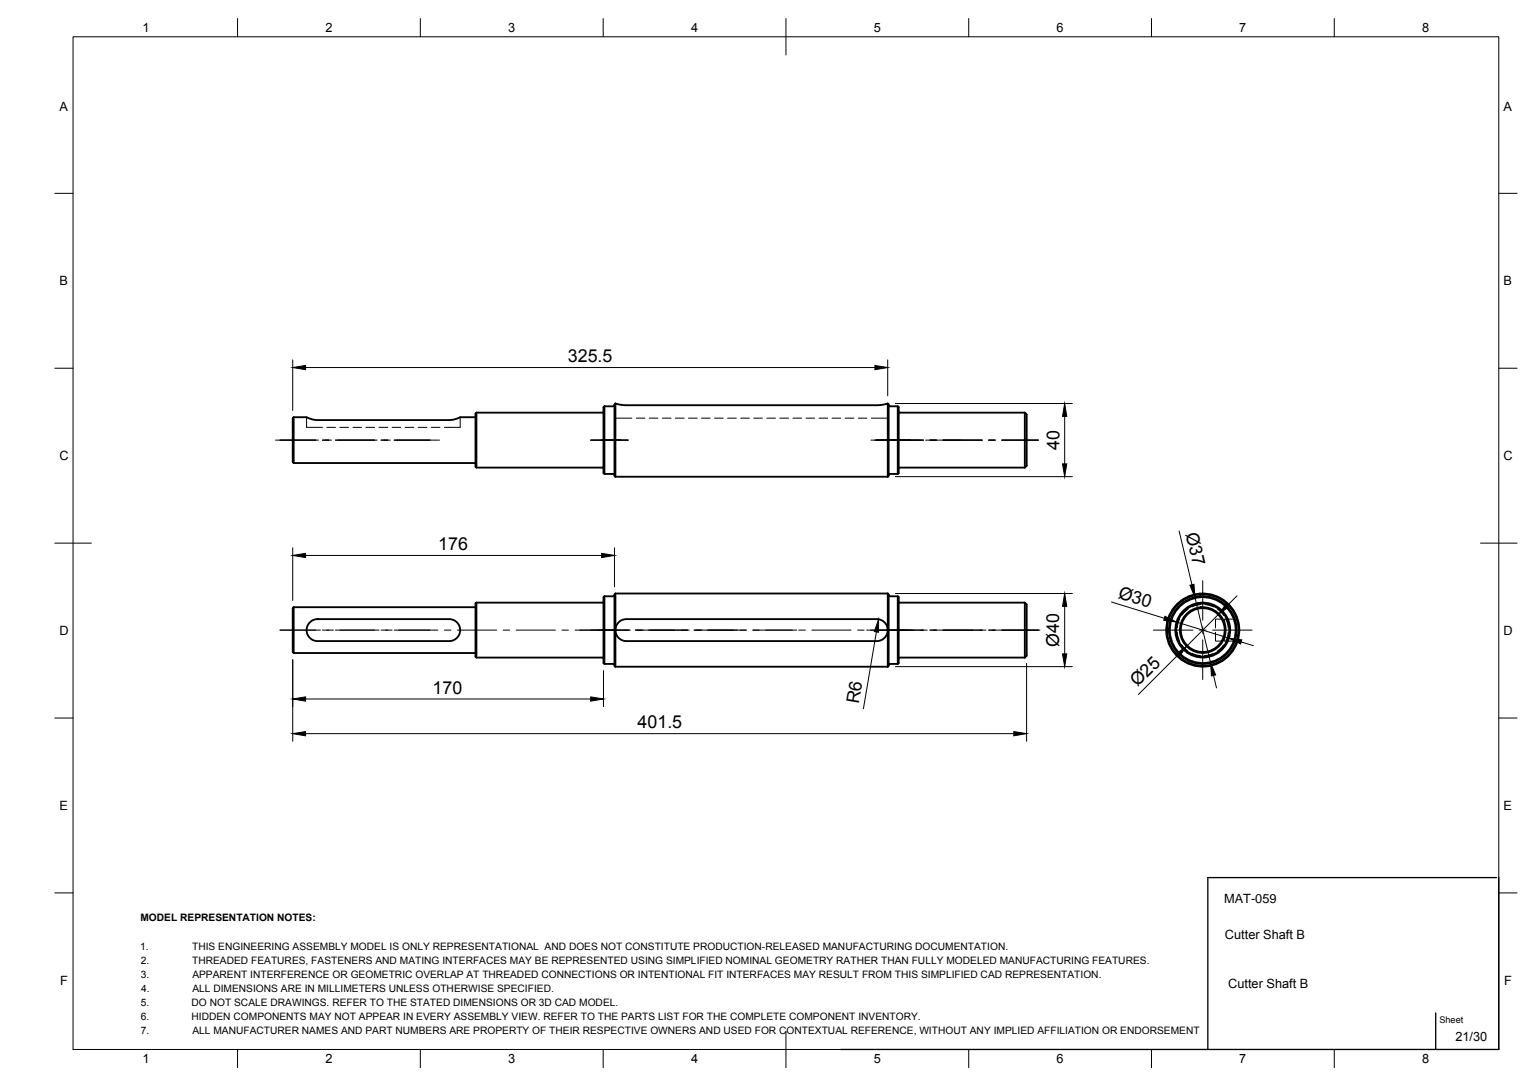
ISO-10303-21;
HEADER;
/* Generated by software containing ST-Developer
 * from STEP Tools, Inc. (www.steptools.com) 
 */

FILE_DESCRIPTION(
/* description */ ('', 'CAx-IF Rec.Pracs.---Representation and Presentation of Product Manufa
cturing Information (PMI)---4.0---2014-10-13'),
/* implementation_level */ '2;1');

FILE_NAME(
/* name */ 'Cutter Shaft B.step',
/* time_stamp */ '2026-10-28T23:00:48+01:00',
/* author */ (''),
/* organization */ (''),
/* preprocessor_version */ 'ST-DEVELOPER v20.2',
/* originating_system */ 'Autodesk Translation Framework v15.17.0.0',
/* authorisation */ '');

FILE_SCHEMA (('AP242_MANAGED_MODEL_BASED_3D_ENGINEERING_MIM_LF { 1 0 10303 442 2 1 4 }'));
ENDSEC;

DATA;
#10=MECHANICAL_DESIGN_GEOMETRIC_PRESENTATION_REPRESENTATION('',(#993),#61811);
#609=CONICAL_SURFACE('',#36036,12.25,0.785398163397429);
#610=CONICAL_SURFACE('',#36043,14.75,0.785398163397442);
#611=CONICAL_SURFACE('',#36058,18.25,0.785398163397442);
#612=CONICAL_SURFACE('',#36079,18.25,0.78539816339745);
#613=CONICAL_SURFACE('',#36085,14.5,0.785398163397445);
#614=CONICAL_SURFACE('',#36103,19.75,0.78539816339745);
#615=CONICAL_SURFACE('',#36104,19.75,0.78539816339745);
#825=B_SPLINE_CURVE_WITH_KNOTS('',3,(#56114,#56115,#56116,#56117,#56118,
#56119,#56120,#56121,#56122,#56123),.UNSPECIFIED.,.F.,.F.,(4,2,2,2,4),(0.910129823137503,
1.1376283823127,1.36512694148791,1.59269329388146,1.82025964627501),
 .UNSPECIFIED.);
#826=B_SPLINE_CURVE_WITH_KNOTS('',3,(#56127,#56128,#56129,#56130,#56131,
#56132,#56133,#56134,#56135,#56136),.UNSPECIFIED.,.F.,.F.,(4,2,2,2,4),(1.82025964627501,
2.04782599866856,2.27539235106211,2.50289091023731,2.73038946941251),
 .UNSPECIFIED.);
#827=B_SPLINE_CURVE_WITH_KNOTS('',3,(#56154,#56155,#56156,#56157,#56158,
#56159,#56160,#56161,#56162,#56163,#56164,#56165,#56166,#56167,#56168,#56169,
#56170,#56171),.UNSPECIFIED.,.F.,.F.,(4,2,2,2,2,2,2,2,4),(-1.84177286144596,
-1.6112902776922,-1.38080769393844,-1.15084706233071,-0.920886430722982,
-0.690925799115252,-0.460965167507522,-0.230482583753761,0.),
 .UNSPECIFIED.);
#828=B_SPLINE_CURVE_WITH_KNOTS('',3,(#56174,#56175,#56176,#56177,#56178,
#56179,#56180,#56181,#56182,#56183,#56184,#56185,#56186,#56187,#56188,#56189,
#56190,#56191),.UNSPECIFIED.,.F.,.F.,(4,2,2,2,2,2,2,2,4),(-3.68354572289192,
-3.45306313913815,-3.22258055538439,-2.99261992377667,-2.76265929216894,
-2.53269866056121,-2.30273802895348,-2.07225544519972,-1.84177286144596),
 .UNSPECIFIED.);
#829=B_SPLINE_CURVE_WITH_KNOTS('',3,(#56285,#56286,#56287,#56288,#56289,
#56290,#56291,#56292,#56293,#56294),.UNSPECIFIED.,.F.,.F.,(4,2,2,2,4),(2.73038946941251,
2.95788802858771,3.18538658776291,3.41295294015646,3.64051929255001),
 .UNSPECIFIED.);
#830=B_SPLINE_CURVE_WITH_KNOTS('',3,(#56306,#56307,#56308,#56309,#56310,
#56311,#56312,#56313,#56314,#56315),.UNSPECIFIED.,.F.,.F.,(4,2,2,2,4),(0.,
0.22756635239355,0.4551327047871,0.682631263962301,0.910129823137503),
 .UNSPECIFIED.);
#902=TOROIDAL_SURFACE('',#36067,15.5,0.5);
#903=TOROIDAL_SURFACE('',#36074,15.5,0.5);
#904=TOROIDAL_SURFACE('',#36098,19.,0.500000000000029);
#905=TOROIDAL_SURFACE('',#36108,19.,0.499999999999998);
#929=SHAPE_REPRESENTATION_RELATIONSHIP('SRR','None',#61989,#954);
#954=ADVANCED_BREP_SHAPE_REPRESENTATION('',(#1032),#61802);
#993=STYLED_ITEM('',(#62156),#1032);
#1032=MANIFOLD_SOLID_BREP('Body1',#33823);
#1380=CYLINDRICAL_SURFACE('',#36033,20.);
#1381=CYLINDRICAL_SURFACE('',#36040,12.5);
#1382=CYLINDRICAL_SURFACE('',#36047,15.);
#1383=CYLINDRICAL_SURFACE('',#36052,5.99999999999999);
#1384=CYLINDRICAL_SURFACE('',#36055,6.00000000000001);
#1385=CYLINDRICAL_SURFACE('',#36064,18.5);
#1386=CYLINDRICAL_SURFACE('',#36071,15.);
#1387=CYLINDRICAL_SURFACE('',#36082,18.5);
#1388=CYLINDRICAL_SURFACE('',#36088,6.);
#1389=CYLINDRICAL_SURFACE('',#36092,6.);
#1390=CYLINDRICAL_SURFACE('',#36095,20.);
#2121=FACE_BOUND('',#7350,.T.);
#2122=FACE_BOUND('',#7355,.T.);
#2123=FACE_BOUND('',#7363,.T.);
#2124=FACE_BOUND('',#7369,.T.);
#2125=FACE_BOUND('',#7382,.T.);
#2126=FACE_BOUND('',#7386,.T.);
#3075=CIRCLE('',#36034,20.);
#3076=CIRCLE('',#36035,20.);
#3077=CIRCLE('',#36037,12.5);
#3078=CIRCLE('',#36038,12.5);
#3079=CIRCLE('',#36039,12.);
#3080=CIRCLE('',#36041,12.5);
#3081=CIRCLE('',#36044,15.);
#3082=CIRCLE('',#36045,15.);
#3083=CIRCLE('',#36046,14.5);
#3084=CIRCLE('',#36048,15.);
#3085=CIRCLE('',#36049,15.);
#3086=CIRCLE('',#36053,5.99999999999999);
#3087=CIRCLE('',#36056,6.00000000000001);
#3088=CIRCLE('',#36059,18.5);
#3089=CIRCLE('',#36060,18.5);
#3090=CIRCLE('',#36061,18.);
#3091=CIRCLE('',#36063,15.5);
#3092=CIRCLE('',#36065,18.5);
#3093=CIRCLE('',#36066,18.5);
#3094=CIRCLE('',#36068,0.5);
#3095=CIRCLE('',#36069,15.);
#3096=CIRCLE('',#36070,15.);
#3097=CIRCLE('',#36072,15.);
#3098=CIRCLE('',#36073,15.);
#3099=CIRCLE('',#36075,0.5);
#3100=CIRCLE('',#36076,15.5);
#3101=CIRCLE('',#36078,18.);
#3102=CIRCLE('',#36080,18.5);
#3103=CIRCLE('',#36081,18.5);
#3104=CIRCLE('',#36083,18.5);
#3105=CIRCLE('',#36084,18.5);
#3106=CIRCLE('',#36086,14.);
#3107=CIRCLE('',#36089,6.);
#3108=CIRCLE('',#36093,6.);
#3109=CIRCLE('',#36096,20.);
#3110=CIRCLE('',#36097,20.);
#3111=CIRCLE('',#36099,19.);
#3112=CIRCLE('',#36100,0.500000000000029);
#3113=CIRCLE('',#36102,19.5);
#3114=CIRCLE('',#36105,19.5);
#3115=CIRCLE('',#36107,19.);
#3116=CIRCLE('',#36109,0.499999999999998);
#5226=FACE_OUTER_BOUND('',#7347,.T.);
#5227=FACE_OUTER_BOUND('',#7348,.T.);
#5228=FACE_OUTER_BOUND('',#7349,.T.);
#5229=FACE_OUTER_BOUND('',#7351,.T.);
#5230=FACE_OUTER_BOUND('',#7352,.T.);
#5231=FACE_OUTER_BOUND('',#7353,.T.);
#5232=FACE_OUTER_BOUND('',#7354,.T.);
#5233=FACE_OUTER_BOUND('',#7356,.T.);
#5234=FACE_OUTER_BOUND('',#7357,.T.);
#5235=FACE_OUTER_BOUND('',#7358,.T.);
#5236=FACE_OUTER_BOUND('',#7359,.T.);
#5237=FACE_OUTER_BOUND('',#7360,.T.);
#5238=FACE_OUTER_BOUND('',#7361,.T.);
#5239=FACE_OUTER_BOUND('',#7362,.T.);
#5240=FACE_OUTER_BOUND('',#7364,.T.);
#5241=FACE_OUTER_BOUND('',#7365,.T.);
#5242=FACE_OUTER_BOUND('',#7366,.T.);
#5243=FACE_OUTER_BOUND('',#7367,.T.);
#5244=FACE_OUTER_BOUND('',#7368,.T.);
#5245=FACE_OUTER_BOUND('',#7370,.T.);
#5246=FACE_OUTER_BOUND('',#7371,.T.);
#5247=FACE_OUTER_BOUND('',#7372,.T.);
#5248=FACE_OUTER_BOUND('',#7373,.T.);
#5249=FACE_OUTER_BOUND('',#7374,.T.);
#5250=FACE_OUTER_BOUND('',#7375,.T.);
#5251=FACE_OUTER_BOUND('',#7376,.T.);
#5252=FACE_OUTER_BOUND('',#7377,.T.);
#5253=FACE_OUTER_BOUND('',#7378,.T.);
#5254=FACE_OUTER_BOUND('',#7379,.T.);
#5255=FACE_OUTER_BOUND('',#7380,.T.);
#5256=FACE_OUTER_BOUND('',#7381,.T.);
#5257=FACE_OUTER_BOUND('',#7383,.T.);
#5258=FACE_OUTER_BOUND('',#7384,.T.);
#5259=FACE_OUTER_BOUND('',#7385,.T.);
#5260=FACE_OUTER_BOUND('',#7387,.T.);
#7347=EDGE_LOOP('',(#26382,#26383,#26384,#26385,#26386,#26387));
#7348=EDGE_LOOP('',(#26388,#26389,#26390,#26391,#26392));
#7349=EDGE_LOOP('',(#26393,#26394,#26395,#26396,#26397));
#7350=EDGE_LOOP('',(#26398,#26399,#26400,#26401));
#7351=EDGE_LOOP('',(#26402));
#7352=EDGE_LOOP('',(#26403,#26404,#26405,#26406,#26407));
#7353=EDGE_LOOP('',(#26408,#26409,#26410,#26411,#26412,#26413));
#7354=EDGE_LOOP('',(#26414));
#7355=EDGE_LOOP('',(#26415));
#7356=EDGE_LOOP('',(#26416,#26417,#26418,#26419));
#7357=EDGE_LOOP('',(#26420,#26421,#26422,#26423));
#7358=EDGE_LOOP('',(#26424,#26425,#26426,#26427));
#7359=EDGE_LOOP('',(#26428,#26429,#26430,#26431));
#7360=EDGE_LOOP('',(#26432,#26433,#26434,#26435));
#7361=EDGE_LOOP('',(#26436,#26437,#26438,#26439,#26440));
#7362=EDGE_LOOP('',(#26441));
#7363=EDGE_LOOP('',(#26442));
#7364=EDGE_LOOP('',(#26443,#26444,#26445,#26446,#26447,#26448));
#7365=EDGE_LOOP('',(#26449,#26450,#26451,#26452,#26453));
#7366=EDGE_LOOP('',(#26454,#26455,#26456,#26457,#26458,#26459));
#7367=EDGE_LOOP('',(#26460,#26461,#26462,#26463,#26464));
#7368=EDGE_LOOP('',(#26465));
#7369=EDGE_LOOP('',(#26466));
#7370=EDGE_LOOP('',(#26467,#26468,#26469,#26470,#26471));
#7371=EDGE_LOOP('',(#26472,#26473,#26474,#26475,#26476,#26477));
#7372=EDGE_LOOP('',(#26478,#26479,#26480,#26481,#26482));
#7373=EDGE_LOOP('',(#26483));
#7374=EDGE_LOOP('',(#26484,#26485,#26486,#26487,#26488));
#7375=EDGE_LOOP('',(#26489,#26490,#26491,#26492));
#7376=EDGE_LOOP('',(#26493,#26494,#26495,#26496));
#7377=EDGE_LOOP('',(#26497,#26498,#26499,#26500,#26501));
#7378=EDGE_LOOP('',(#26502,#26503,#26504,#26505));
#7379=EDGE_LOOP('',(#26506,#26507,#26508,#26509,#26510,#26511));
#7380=EDGE_LOOP('',(#26512,#26513,#26514,#26515,#26516));
#7381=EDGE_LOOP('',(#26517));
#7382=EDGE_LOOP('',(#26518));
#7383=EDGE_LOOP('',(#26519,#26520,#26521,#26522,#26523));
#7384=EDGE_LOOP('',(#26524,#26525,#26526,#26527,#26528));
#7385=EDGE_LOOP('',(#26529));
#7386=EDGE_LOOP('',(#26530));
#7387=EDGE_LOOP('',(#26531,#26532,#26533,#26534,#26535));
#9784=LINE('',#56110,#12331);
#9785=LINE('',#56125,#12332);
#9786=LINE('',#56144,#12333);
#9787=LINE('',#56148,#12334);
#9788=LINE('',#56152,#12335);
#9789=LINE('',#56173,#12336);
#9790=LINE('',#56199,#12337);
#9791=LINE('',#56203,#12338);
#9792=LINE('',#56210,#12339);
#9793=LINE('',#56212,#12340);
#9794=LINE('',#56213,#12341);
#9795=LINE('',#56217,#12342);
#9796=LINE('',#56220,#12343);
#9797=LINE('',#56221,#12344);
#9798=LINE('',#56231,#12345);
#9799=LINE('',#56240,#12346);
#9800=LINE('',#56250,#12347);
#9801=LINE('',#56266,#12348);
#9802=LINE('',#56269,#12349);
#9803=LINE('',#56275,#12350);
#9804=LINE('',#56280,#12351);
#9805=LINE('',#56284,#12352);
#9806=LINE('',#56297,#12353);
#9807=LINE('',#56299,#12354);
#9808=LINE('',#56300,#12355);
#9809=LINE('',#56303,#12356);
#9810=LINE('',#56304,#12357);
#9811=LINE('',#56329,#12358);
#9812=LINE('',#56332,#12359);
#12331=VECTOR('',#43448,20.);
#12332=VECTOR('',#43451,10.);
#12333=VECTOR('',#43460,12.25);
#12334=VECTOR('',#43465,12.5);
#12335=VECTOR('',#43468,10.);
#12336=VECTOR('',#43469,10.);
#12337=VECTOR('',#43478,14.75);
#12338=VECTOR('',#43483,15.);
#12339=VECTOR('',#43492,10.);
#12340=VECTOR('',#43493,10.);
#12341=VECTOR('',#43494,10.);
#12342=VECTOR('',#43499,10.);
#12343=VECTOR('',#43502,10.);
#12344=VECTOR('',#43503,10.);
#12345=VECTOR('',#43516,18.25);
#12346=VECTOR('',#43527,18.5);
#12347=VECTOR('',#43540,15.);
#12348=VECTOR('',#43561,18.25);
#12349=VECTOR('',#43564,18.5);
#12350=VECTOR('',#43571,14.5);
#12351=VECTOR('',#43578,10.);
#12352=VECTOR('',#43581,10.);
#12353=VECTOR('',#43584,10.);
#12354=VECTOR('',#43585,10.);
#12355=VECTOR('',#43586,10.);
#12356=VECTOR('',#43589,10.);
#12357=VECTOR('',#43590,10.);
#12358=VECTOR('',#43615,19.75);
#12359=VECTOR('',#43618,19.75);
#15047=VERTEX_POINT('',#56108);
#15048=VERTEX_POINT('',#56109);
#15049=VERTEX_POINT('',#56111);
#15050=VERTEX_POINT('',#56113);
#15051=VERTEX_POINT('',#56124);
#15052=VERTEX_POINT('',#56126);
#15053=VERTEX_POINT('',#56139);
#15054=VERTEX_POINT('',#56140);
#15055=VERTEX_POINT('',#56143);
#15056=VERTEX_POINT('',#56147);
#15057=VERTEX_POINT('',#56150);
#15058=VERTEX_POINT('',#56151);
#15059=VERTEX_POINT('',#56153);
#15060=VERTEX_POINT('',#56172);
#15061=VERTEX_POINT('',#56194);
#15062=VERTEX_POINT('',#56195);
#15063=VERTEX_POINT('',#56198);
#15064=VERTEX_POINT('',#56202);
#15065=VERTEX_POINT('',#56204);
#15066=VERTEX_POINT('',#56209);
#15067=VERTEX_POINT('',#56211);
#15068=VERTEX_POINT('',#56215);
#15069=VERTEX_POINT('',#56219);
#15070=VERTEX_POINT('',#56226);
#15071=VERTEX_POINT('',#56227);
#15072=VERTEX_POINT('',#56230);
#15073=VERTEX_POINT('',#56234);
#15074=VERTEX_POINT('',#56237);
#15075=VERTEX_POINT('',#56238);
#15076=VERTEX_POINT('',#56243);
#15077=VERTEX_POINT('',#56245);
#15078=VERTEX_POINT('',#56249);
#15079=VERTEX_POINT('',#56251);
#15080=VERTEX_POINT('',#56255);
#15081=VERTEX_POINT('',#56259);
#15082=VERTEX_POINT('',#56262);
#15083=VERTEX_POINT('',#56263);
#15084=VERTEX_POINT('',#56268);
#15085=VERTEX_POINT('',#56270);
#15086=VERTEX_POINT('',#56274);
#15087=VERTEX_POINT('',#56279);
#15088=VERTEX_POINT('',#56281);
#15089=VERTEX_POINT('',#56283);
#15090=VERTEX_POINT('',#56296);
#15091=VERTEX_POINT('',#56298);
#15092=VERTEX_POINT('',#56302);
#15093=VERTEX_POINT('',#56322);
#15094=VERTEX_POINT('',#56326);
#15095=VERTEX_POINT('',#56331);
#15096=VERTEX_POINT('',#56335);
#19093=EDGE_CURVE('',#15047,#15048,#9784,.T.);
#19094=EDGE_CURVE('',#15049,#15047,#3075,.T.);
#19095=EDGE_CURVE('',#15049,#15050,#825,.T.);
#19096=EDGE_CURVE('',#15050,#15051,#9785,.T.);
#19097=EDGE_CURVE('',#15051,#15052,#826,.T.);
#19098=EDGE_CURVE('',#15052,#15048,#3076,.T.);
#19099=EDGE_CURVE('',#15053,#15054,#3077,.T.);
#19100=EDGE_CURVE('',#15054,#15053,#3078,.T.);
#19101=EDGE_CURVE('',#15053,#15055,#9786,.T.);
#19102=EDGE_CURVE('',#15055,#15055,#3079,.T.);
#19103=EDGE_CURVE('',#15054,#15056,#9787,.T.);
#19104=EDGE_CURVE('',#15056,#15056,#3080,.T.);
#19105=EDGE_CURVE('',#15057,#15058,#9788,.T.);
#19106=EDGE_CURVE('',#15058,#15059,#827,.T.);
#19107=EDGE_CURVE('',#15059,#15060,#9789,.T.);
#19108=EDGE_CURVE('',#15060,#15057,#828,.T.);
#19109=EDGE_CURVE('',#15061,#15062,#3081,.T.);
#19110=EDGE_CURVE('',#15062,#15061,#3082,.T.);
#19111=EDGE_CURVE('',#15061,#15063,#9790,.T.);
#19112=EDGE_CURVE('',#15063,#15063,#3083,.T.);
#19113=EDGE_CURVE('',#15062,#15064,#9791,.T.);
#19114=EDGE_CURVE('',#15065,#15064,#3084,.T.);
#19115=EDGE_CURVE('',#15064,#15065,#3085,.T.);
#19116=EDGE_CURVE('',#15059,#15066,#9792,.T.);
#19117=EDGE_CURVE('',#15066,#15067,#9793,.T.);
#19118=EDGE_CURVE('',#15060,#15067,#9794,.T.);
#19119=EDGE_CURVE('',#15067,#15068,#3086,.T.);
#19120=EDGE_CURVE('',#15057,#15068,#9795,.T.);
#19121=EDGE_CURVE('',#15068,#15069,#9796,.T.);
#19122=EDGE_CURVE('',#15058,#15069,#9797,.T.);
#19123=EDGE_CURVE('',#15069,#15066,#3087,.T.);
#19124=EDGE_CURVE('',#15070,#15071,#3088,.T.);
#19125=EDGE_CURVE('',#15071,#15070,#3089,.T.);
#19126=EDGE_CURVE('',#15070,#15072,#9798,.T.);
#19127=EDGE_CURVE('',#15072,#15072,#3090,.T.);
#19128=EDGE_CURVE('',#15073,#15073,#3091,.T.);
#19129=EDGE_CURVE('',#15074,#15075,#3092,.T.);
#19130=EDGE_CURVE('',#15074,#15071,#9799,.T.);
#19131=EDGE_CURVE('',#15075,#15074,#3093,.T.);
#19132=EDGE_CURVE('',#15073,#15076,#3094,.T.);
#19133=EDGE_CURVE('',#15076,#15077,#3095,.T.);
#19134=EDGE_CURVE('',#15077,#15076,#3096,.T.);
#19135=EDGE_CURVE('',#15077,#15078,#9800,.T.);
#19136=EDGE_CURVE('',#15079,#15078,#3097,.T.);
#19137=EDGE_CURVE('',#15078,#15079,#3098,.T.);
#19138=EDGE_CURVE('',#15065,#15080,#3099,.T.);
#19139=EDGE_CURVE('',#15080,#15080,#3100,.T.);
#19140=EDGE_CURVE('',#15081,#15081,#3101,.T.);
#19141=EDGE_CURVE('',#15082,#15083,#3102,.T.);
#19142=EDGE_CURVE('',#15083,#15082,#3103,.T.);
#19143=EDGE_CURVE('',#15082,#15081,#9801,.T.);
#19144=EDGE_CURVE('',#15083,#15084,#9802,.T.);
#19145=EDGE_CURVE('',#15084,#15085,#3104,.T.);
#19146=EDGE_CURVE('',#15085,#15084,#3105,.T.);
#19147=EDGE_CURVE('',#15079,#15086,#9803,.T.);
#19148=EDGE_CURVE('',#15086,#15086,#3106,.T.);
#19149=EDGE_CURVE('',#15051,#15087,#9804,.T.);
#19150=EDGE_CURVE('',#15087,#15088,#3107,.T.);
#19151=EDGE_CURVE('',#15089,#15088,#9805,.T.);
#19152=EDGE_CURVE('',#15052,#15089,#829,.T.);
#19153=EDGE_CURVE('',#15089,#15090,#9806,.T.);
#19154=EDGE_CURVE('',#15088,#15091,#9807,.T.);
#19155=EDGE_CURVE('',#15090,#15091,#9808,.T.);
#19156=EDGE_CURVE('',#15050,#15092,#9809,.T.);
#19157=EDGE_CURVE('',#15092,#15087,#9810,.T.);
#19158=EDGE_CURVE('',#15090,#15049,#830,.T.);
#19159=EDGE_CURVE('',#15091,#15092,#3108,.T.);
#19160=EDGE_CURVE('',#15048,#15052,#3109,.T.);
#19161=EDGE_CURVE('',#15047,#15049,#3110,.T.);
#19162=EDGE_CURVE('',#15093,#15093,#3111,.T.);
#19163=EDGE_CURVE('',#15093,#15075,#3112,.T.);
#19164=EDGE_CURVE('',#15094,#15094,#3113,.T.);
#19165=EDGE_CURVE('',#15048,#15094,#9811,.T.);
#19166=EDGE_CURVE('',#15047,#15095,#9812,.T.);
#19167=EDGE_CURVE('',#15095,#15095,#3114,.T.);
#19168=EDGE_CURVE('',#15096,#15096,#3115,.T.);
#19169=EDGE_CURVE('',#15085,#15096,#3116,.T.);
#26382=ORIENTED_EDGE('',*,*,#19093,.F.);
#26383=ORIENTED_EDGE('',*,*,#19094,.F.);
#26384=ORIENTED_EDGE('',*,*,#19095,.T.);
#26385=ORIENTED_EDGE('',*,*,#19096,.T.);
#26386=ORIENTED_EDGE('',*,*,#19097,.T.);
#26387=ORIENTED_EDGE('',*,*,#19098,.T.);
#26388=ORIENTED_EDGE('',*,*,#19099,.T.);
#26389=ORIENTED_EDGE('',*,*,#19100,.T.);
#26390=ORIENTED_EDGE('',*,*,#19101,.T.);
#26391=ORIENTED_EDGE('',*,*,#19102,.T.);
#26392=ORIENTED_EDGE('',*,*,#19101,.F.);
#26393=ORIENTED_EDGE('',*,*,#19099,.F.);
#26394=ORIENTED_EDGE('',*,*,#19100,.F.);
#26395=ORIENTED_EDGE('',*,*,#19103,.T.);
#26396=ORIENTED_EDGE('',*,*,#19104,.T.);
#26397=ORIENTED_EDGE('',*,*,#19103,.F.);
#26398=ORIENTED_EDGE('',*,*,#19105,.T.);
#26399=ORIENTED_EDGE('',*,*,#19106,.T.);
#26400=ORIENTED_EDGE('',*,*,#19107,.T.);
#26401=ORIENTED_EDGE('',*,*,#19108,.T.);
#26402=ORIENTED_EDGE('',*,*,#19102,.F.);
#26403=ORIENTED_EDGE('',*,*,#19109,.T.);
#26404=ORIENTED_EDGE('',*,*,#19110,.T.);
#26405=ORIENTED_EDGE('',*,*,#19111,.T.);
#26406=ORIENTED_EDGE('',*,*,#19112,.T.);
#26407=ORIENTED_EDGE('',*,*,#19111,.F.);
#26408=ORIENTED_EDGE('',*,*,#19109,.F.);
#26409=ORIENTED_EDGE('',*,*,#19110,.F.);
#26410=ORIENTED_EDGE('',*,*,#19113,.T.);
#26411=ORIENTED_EDGE('',*,*,#19114,.F.);
#26412=ORIENTED_EDGE('',*,*,#19115,.F.);
#26413=ORIENTED_EDGE('',*,*,#19113,.F.);
#26414=ORIENTED_EDGE('',*,*,#19112,.F.);
#26415=ORIENTED_EDGE('',*,*,#19104,.F.);
#26416=ORIENTED_EDGE('',*,*,#19107,.F.);
#26417=ORIENTED_EDGE('',*,*,#19116,.T.);
#26418=ORIENTED_EDGE('',*,*,#19117,.T.);
#26419=ORIENTED_EDGE('',*,*,#19118,.F.);
#26420=ORIENTED_EDGE('',*,*,#19108,.F.);
#26421=ORIENTED_EDGE('',*,*,#19118,.T.);
#26422=ORIENTED_EDGE('',*,*,#19119,.T.);
#26423=ORIENTED_EDGE('',*,*,#19120,.F.);
#26424=ORIENTED_EDGE('',*,*,#19105,.F.);
#26425=ORIENTED_EDGE('',*,*,#19120,.T.);
#26426=ORIENTED_EDGE('',*,*,#19121,.T.);
#26427=ORIENTED_EDGE('',*,*,#19122,.F.);
#26428=ORIENTED_EDGE('',*,*,#19106,.F.);
#26429=ORIENTED_EDGE('',*,*,#19122,.T.);
#26430=ORIENTED_EDGE('',*,*,#19123,.T.);
#26431=ORIENTED_EDGE('',*,*,#19116,.F.);
#26432=ORIENTED_EDGE('',*,*,#19123,.F.);
#26433=ORIENTED_EDGE('',*,*,#19121,.F.);
#26434=ORIENTED_EDGE('',*,*,#19119,.F.);
#26435=ORIENTED_EDGE('',*,*,#19117,.F.);
#26436=ORIENTED_EDGE('',*,*,#19124,.T.);
#26437=ORIENTED_EDGE('',*,*,#19125,.T.);
#26438=ORIENTED_EDGE('',*,*,#19126,.T.);
#26439=ORIENTED_EDGE('',*,*,#19127,.T.);
#26440=ORIENTED_EDGE('',*,*,#19126,.F.);
#26441=ORIENTED_EDGE('',*,*,#19127,.F.);
#26442=ORIENTED_EDGE('',*,*,#19128,.F.);
#26443=ORIENTED_EDGE('',*,*,#19129,.F.);
#26444=ORIENTED_EDGE('',*,*,#19130,.T.);
#26445=ORIENTED_EDGE('',*,*,#19124,.F.);
#26446=ORIENTED_EDGE('',*,*,#19125,.F.);
#26447=ORIENTED_EDGE('',*,*,#19130,.F.);
#26448=ORIENTED_EDGE('',*,*,#19131,.F.);
#26449=ORIENTED_EDGE('',*,*,#19128,.T.);
#26450=ORIENTED_EDGE('',*,*,#19132,.T.);
#26451=ORIENTED_EDGE('',*,*,#19133,.T.);
#26452=ORIENTED_EDGE('',*,*,#19134,.T.);
#26453=ORIENTED_EDGE('',*,*,#19132,.F.);
#26454=ORIENTED_EDGE('',*,*,#19134,.F.);
#26455=ORIENTED_EDGE('',*,*,#19135,.T.);
#26456=ORIENTED_EDGE('',*,*,#19136,.F.);
#26457=ORIENTED_EDGE('',*,*,#19137,.F.);
#26458=ORIENTED_EDGE('',*,*,#19135,.F.);
#26459=ORIENTED_EDGE('',*,*,#19133,.F.);
#26460=ORIENTED_EDGE('',*,*,#19114,.T.);
#26461=ORIENTED_EDGE('',*,*,#19115,.T.);
#26462=ORIENTED_EDGE('',*,*,#19138,.T.);
#26463=ORIENTED_EDGE('',*,*,#19139,.T.);
#26464=ORIENTED_EDGE('',*,*,#19138,.F.);
#26465=ORIENTED_EDGE('',*,*,#19140,.F.);
#26466=ORIENTED_EDGE('',*,*,#19139,.F.);
#26467=ORIENTED_EDGE('',*,*,#19141,.T.);
#26468=ORIENTED_EDGE('',*,*,#19142,.T.);
#26469=ORIENTED_EDGE('',*,*,#19143,.T.);
#26470=ORIENTED_EDGE('',*,*,#19140,.T.);
#26471=ORIENTED_EDGE('',*,*,#19143,.F.);
#26472=ORIENTED_EDGE('',*,*,#19141,.F.);
#26473=ORIENTED_EDGE('',*,*,#19142,.F.);
#26474=ORIENTED_EDGE('',*,*,#19144,.T.);
#26475=ORIENTED_EDGE('',*,*,#19145,.T.);
#26476=ORIENTED_EDGE('',*,*,#19146,.T.);
#26477=ORIENTED_EDGE('',*,*,#19144,.F.);
#26478=ORIENTED_EDGE('',*,*,#19136,.T.);
#26479=ORIENTED_EDGE('',*,*,#19137,.T.);
#26480=ORIENTED_EDGE('',*,*,#19147,.T.);
#26481=ORIENTED_EDGE('',*,*,#19148,.T.);
#26482=ORIENTED_EDGE('',*,*,#19147,.F.);
#26483=ORIENTED_EDGE('',*,*,#19148,.F.);
#26484=ORIENTED_EDGE('',*,*,#19097,.F.);
#26485=ORIENTED_EDGE('',*,*,#19149,.T.);
#26486=ORIENTED_EDGE('',*,*,#19150,.T.);
#26487=ORIENTED_EDGE('',*,*,#19151,.F.);
#26488=ORIENTED_EDGE('',*,*,#19152,.F.);
#26489=ORIENTED_EDGE('',*,*,#19153,.F.);
#26490=ORIENTED_EDGE('',*,*,#19151,.T.);
#26491=ORIENTED_EDGE('',*,*,#19154,.T.);
#26492=ORIENTED_EDGE('',*,*,#19155,.F.);
#26493=ORIENTED_EDGE('',*,*,#19096,.F.);
#26494=ORIENTED_EDGE('',*,*,#19156,.T.);
#26495=ORIENTED_EDGE('',*,*,#19157,.T.);
#26496=ORIENTED_EDGE('',*,*,#19149,.F.);
#26497=ORIENTED_EDGE('',*,*,#19095,.F.);
#26498=ORIENTED_EDGE('',*,*,#19158,.F.);
#26499=ORIENTED_EDGE('',*,*,#19155,.T.);
#26500=ORIENTED_EDGE('',*,*,#19159,.T.);
#26501=ORIENTED_EDGE('',*,*,#19156,.F.);
#26502=ORIENTED_EDGE('',*,*,#19150,.F.);
#26503=ORIENTED_EDGE('',*,*,#19157,.F.);
#26504=ORIENTED_EDGE('',*,*,#19159,.F.);
#26505=ORIENTED_EDGE('',*,*,#19154,.F.);
#26506=ORIENTED_EDGE('',*,*,#19093,.T.);
#26507=ORIENTED_EDGE('',*,*,#19160,.T.);
#26508=ORIENTED_EDGE('',*,*,#19152,.T.);
#26509=ORIENTED_EDGE('',*,*,#19153,.T.);
#26510=ORIENTED_EDGE('',*,*,#19158,.T.);
#26511=ORIENTED_EDGE('',*,*,#19161,.F.);
#26512=ORIENTED_EDGE('',*,*,#19162,.F.);
#26513=ORIENTED_EDGE('',*,*,#19163,.T.);
#26514=ORIENTED_EDGE('',*,*,#19131,.T.);
#26515=ORIENTED_EDGE('',*,*,#19129,.T.);
#26516=ORIENTED_EDGE('',*,*,#19163,.F.);
#26517=ORIENTED_EDGE('',*,*,#19164,.F.);
#26518=ORIENTED_EDGE('',*,*,#19162,.T.);
#26519=ORIENTED_EDGE('',*,*,#19098,.F.);
#26520=ORIENTED_EDGE('',*,*,#19160,.F.);
#26521=ORIENTED_EDGE('',*,*,#19165,.T.);
#26522=ORIENTED_EDGE('',*,*,#19164,.T.);
#26523=ORIENTED_EDGE('',*,*,#19165,.F.);
#26524=ORIENTED_EDGE('',*,*,#19094,.T.);
#26525=ORIENTED_EDGE('',*,*,#19166,.T.);
#26526=ORIENTED_EDGE('',*,*,#19167,.F.);
#26527=ORIENTED_EDGE('',*,*,#19166,.F.);
#26528=ORIENTED_EDGE('',*,*,#19161,.T.);
#26529=ORIENTED_EDGE('',*,*,#19167,.T.);
#26530=ORIENTED_EDGE('',*,*,#19168,.F.);
#26531=ORIENTED_EDGE('',*,*,#19145,.F.);
#26532=ORIENTED_EDGE('',*,*,#19146,.F.);
#26533=ORIENTED_EDGE('',*,*,#19169,.T.);
#26534=ORIENTED_EDGE('',*,*,#19168,.T.);
#26535=ORIENTED_EDGE('',*,*,#19169,.F.);
#31637=PLANE('',#36042);
#31638=PLANE('',#36050);
#31639=PLANE('',#36051);
#31640=PLANE('',#36054);
#31641=PLANE('',#36057);
#31642=PLANE('',#36062);
#31643=PLANE('',#36077);
#31644=PLANE('',#36087);
#31645=PLANE('',#36090);
#31646=PLANE('',#36091);
#31647=PLANE('',#36094);
#31648=PLANE('',#36101);
#31649=PLANE('',#36106);
#32907=ADVANCED_FACE('',(#5226),#1380,.T.);
#32908=ADVANCED_FACE('',(#5227),#609,.T.);
#32909=ADVANCED_FACE('',(#5228,#2121),#1381,.T.);
#32910=ADVANCED_FACE('',(#5229),#31637,.T.);
#32911=ADVANCED_FACE('',(#5230),#610,.T.);
#32912=ADVANCED_FACE('',(#5231),#1382,.T.);
#32913=ADVANCED_FACE('',(#5232,#2122),#31638,.T.);
#32914=ADVANCED_FACE('',(#5233),#31639,.F.);
#32915=ADVANCED_FACE('',(#5234),#1383,.F.);
#32916=ADVANCED_FACE('',(#5235),#31640,.F.);
#32917=ADVANCED_FACE('',(#5236),#1384,.F.);
#32918=ADVANCED_FACE('',(#5237),#31641,.F.);
#32919=ADVANCED_FACE('',(#5238),#611,.T.);
#32920=ADVANCED_FACE('',(#5239,#2123),#31642,.T.);
#32921=ADVANCED_FACE('',(#5240),#1385,.T.);
#32922=ADVANCED_FACE('',(#5241),#902,.F.);
#32923=ADVANCED_FACE('',(#5242),#1386,.T.);
#32924=ADVANCED_FACE('',(#5243),#903,.F.);
#32925=ADVANCED_FACE('',(#5244,#2124),#31643,.T.);
#32926=ADVANCED_FACE('',(#5245),#612,.T.);
#32927=ADVANCED_FACE('',(#5246),#1387,.T.);
#32928=ADVANCED_FACE('',(#5247),#613,.T.);
#32929=ADVANCED_FACE('',(#5248),#31644,.T.);
#32930=ADVANCED_FACE('',(#5249),#1388,.F.);
#32931=ADVANCED_FACE('',(#5250),#31645,.F.);
#32932=ADVANCED_FACE('',(#5251),#31646,.F.);
#32933=ADVANCED_FACE('',(#5252),#1389,.F.);
#32934=ADVANCED_FACE('',(#5253),#31647,.T.);
#32935=ADVANCED_FACE('',(#5254),#1390,.T.);
#32936=ADVANCED_FACE('',(#5255),#904,.F.);
#32937=ADVANCED_FACE('',(#5256,#2125),#31648,.T.);
#32938=ADVANCED_FACE('',(#5257),#614,.T.);
#32939=ADVANCED_FACE('',(#5258),#615,.T.);
#32940=ADVANCED_FACE('',(#5259,#2126),#31649,.T.);
#32941=ADVANCED_FACE('',(#5260),#905,.F.);
#33823=CLOSED_SHELL('',(#32907,#32908,#32909,#32910,#32911,#32912,#32913,
#32914,#32915,#32916,#32917,#32918,#32919,#32920,#32921,#32922,#32923,#32924,
#32925,#32926,#32927,#32928,#32929,#32930,#32931,#32932,#32933,#32934,#32935,
#32936,#32937,#32938,#32939,#32940,#32941));
#36032=AXIS2_PLACEMENT_3D('',#56106,#43444,#43445);
#36033=AXIS2_PLACEMENT_3D('',#56107,#43446,#43447);
#36034=AXIS2_PLACEMENT_3D('',#56112,#43449,#43450);
#36035=AXIS2_PLACEMENT_3D('',#56137,#43452,#43453);
#36036=AXIS2_PLACEMENT_3D('',#56138,#43454,#43455);
#36037=AXIS2_PLACEMENT_3D('',#56141,#43456,#43457);
#36038=AXIS2_PLACEMENT_3D('',#56142,#43458,#43459);
#36039=AXIS2_PLACEMENT_3D('',#56145,#43461,#43462);
#36040=AXIS2_PLACEMENT_3D('',#56146,#43463,#43464);
#36041=AXIS2_PLACEMENT_3D('',#56149,#43466,#43467);
#36042=AXIS2_PLACEMENT_3D('',#56192,#43470,#43471);
#36043=AXIS2_PLACEMENT_3D('',#56193,#43472,#43473);
#36044=AXIS2_PLACEMENT_3D('',#56196,#43474,#43475);
#36045=AXIS2_PLACEMENT_3D('',#56197,#43476,#43477);
#36046=AXIS2_PLACEMENT_3D('',#56200,#43479,#43480);
#36047=AXIS2_PLACEMENT_3D('',#56201,#43481,#43482);
#36048=AXIS2_PLACEMENT_3D('',#56205,#43484,#43485);
#36049=AXIS2_PLACEMENT_3D('',#56206,#43486,#43487);
#36050=AXIS2_PLACEMENT_3D('',#56207,#43488,#43489);
#36051=AXIS2_PLACEMENT_3D('',#56208,#43490,#43491);
#36052=AXIS2_PLACEMENT_3D('',#56214,#43495,#43496);
#36053=AXIS2_PLACEMENT_3D('',#56216,#43497,#43498);
#36054=AXIS2_PLACEMENT_3D('',#56218,#43500,#43501);
#36055=AXIS2_PLACEMENT_3D('',#56222,#43504,#43505);
#36056=AXIS2_PLACEMENT_3D('',#56223,#43506,#43507);
#36057=AXIS2_PLACEMENT_3D('',#56224,#43508,#43509);
#36058=AXIS2_PLACEMENT_3D('',#56225,#43510,#43511);
#36059=AXIS2_PLACEMENT_3D('',#56228,#43512,#43513);
#36060=AXIS2_PLACEMENT_3D('',#56229,#43514,#43515);
#36061=AXIS2_PLACEMENT_3D('',#56232,#43517,#43518);
#36062=AXIS2_PLACEMENT_3D('',#56233,#43519,#43520);
#36063=AXIS2_PLACEMENT_3D('',#56235,#43521,#43522);
#36064=AXIS2_PLACEMENT_3D('',#56236,#43523,#43524);
#36065=AXIS2_PLACEMENT_3D('',#56239,#43525,#43526);
#36066=AXIS2_PLACEMENT_3D('',#56241,#43528,#43529);
#36067=AXIS2_PLACEMENT_3D('',#56242,#43530,#43531);
#36068=AXIS2_PLACEMENT_3D('',#56244,#43532,#43533);
#36069=AXIS2_PLACEMENT_3D('',#56246,#43534,#43535);
#36070=AXIS2_PLACEMENT_3D('',#56247,#43536,#43537);
#36071=AXIS2_PLACEMENT_3D('',#56248,#43538,#43539);
#36072=AXIS2_PLACEMENT_3D('',#56252,#43541,#43542);
#36073=AXIS2_PLACEMENT_3D('',#56253,#43543,#43544);
#36074=AXIS2_PLACEMENT_3D('',#56254,#43545,#43546);
#36075=AXIS2_PLACEMENT_3D('',#56256,#43547,#43548);
#36076=AXIS2_PLACEMENT_3D('',#56257,#43549,#43550);
#36077=AXIS2_PLACEMENT_3D('',#56258,#43551,#43552);
#36078=AXIS2_PLACEMENT_3D('',#56260,#43553,#43554);
#36079=AXIS2_PLACEMENT_3D('',#56261,#43555,#43556);
#36080=AXIS2_PLACEMENT_3D('',#56264,#43557,#43558);
#36081=AXIS2_PLACEMENT_3D('',#56265,#43559,#43560);
#36082=AXIS2_PLACEMENT_3D('',#56267,#43562,#43563);
#36083=AXIS2_PLACEMENT_3D('',#56271,#43565,#43566);
#36084=AXIS2_PLACEMENT_3D('',#56272,#43567,#43568);
#36085=AXIS2_PLACEMENT_3D('',#56273,#43569,#43570);
#36086=AXIS2_PLACEMENT_3D('',#56276,#43572,#43573);
#36087=AXIS2_PLACEMENT_3D('',#56277,#43574,#43575);
#36088=AXIS2_PLACEMENT_3D('',#56278,#43576,#43577);
#36089=AXIS2_PLACEMENT_3D('',#56282,#43579,#43580);
#36090=AXIS2_PLACEMENT_3D('',#56295,#43582,#43583);
#36091=AXIS2_PLACEMENT_3D('',#56301,#43587,#43588);
#36092=AXIS2_PLACEMENT_3D('',#56305,#43591,#43592);
#36093=AXIS2_PLACEMENT_3D('',#56316,#43593,#43594);
#36094=AXIS2_PLACEMENT_3D('',#56317,#43595,#43596);
#36095=AXIS2_PLACEMENT_3D('',#56318,#43597,#43598);
#36096=AXIS2_PLACEMENT_3D('',#56319,#43599,#43600);
#36097=AXIS2_PLACEMENT_3D('',#56320,#43601,#43602);
#36098=AXIS2_PLACEMENT_3D('',#56321,#43603,#43604);
#36099=AXIS2_PLACEMENT_3D('',#56323,#43605,#43606);
#36100=AXIS2_PLACEMENT_3D('',#56324,#43607,#43608);
#36101=AXIS2_PLACEMENT_3D('',#56325,#43609,#43610);
#36102=AXIS2_PLACEMENT_3D('',#56327,#43611,#43612);
#36103=AXIS2_PLACEMENT_3D('',#56328,#43613,#43614);
#36104=AXIS2_PLACEMENT_3D('',#56330,#43616,#43617);
#36105=AXIS2_PLACEMENT_3D('',#56333,#43619,#43620);
#36106=AXIS2_PLACEMENT_3D('',#56334,#43621,#43622);
#36107=AXIS2_PLACEMENT_3D('',#56336,#43623,#43624);
#36108=AXIS2_PLACEMENT_3D('',#56337,#43625,#43626);
#36109=AXIS2_PLACEMENT_3D('',#56338,#43627,#43628);
#43444=DIRECTION('axis',(0.,0.,1.));
#43445=DIRECTION('refdir',(1.,0.,0.));
#43446=DIRECTION('center_axis',(4.88578148594761E-16,1.,1.17579033359749E-15));
#43447=DIRECTION('ref_axis',(0.0779446090567885,1.13413118345969E-15,-0.996957691137886));
#43448=DIRECTION('',(-4.88578148594761E-16,-1.,-1.17579033359749E-15));
#43449=DIRECTION('center_axis',(4.88578148594761E-16,1.,1.17579033359749E-15));
#43450=DIRECTION('ref_axis',(0.996957691137886,-5.78738260848463E-16,0.0779446090567885));
#43451=DIRECTION('',(-4.88578148594761E-16,-1.,-1.17579033359749E-15));
#43452=DIRECTION('center_axis',(4.88578148594761E-16,1.,1.17579033359749E-15));
#43453=DIRECTION('ref_axis',(0.996957691137886,-5.78738260848463E-16,0.0779446090567885));
#43454=DIRECTION('center_axis',(-4.88578148594761E-16,-1.,-1.17579033359749E-15));
#43455=DIRECTION('ref_axis',(-0.0779446090567885,-1.13413118345969E-15,
0.996957691137886));
#43456=DIRECTION('center_axis',(4.88578148594761E-16,1.,1.17579033359749E-15));
#43457=DIRECTION('ref_axis',(-0.0779446090567885,-1.13413118345969E-15,
0.996957691137886));
#43458=DIRECTION('center_axis',(4.88578148594761E-16,1.,1.17579033359749E-15));
#43459=DIRECTION('ref_axis',(-0.0779446090567885,-1.13413118345969E-15,
0.996957691137886));
#43460=DIRECTION('',(-0.0551151616209882,0.70710678118656,0.70495554395967));
#43461=DIRECTION('center_axis',(-4.88578148594761E-16,-1.,-1.17579033359749E-15));
#43462=DIRECTION('ref_axis',(-0.0779446090567885,-1.13413118345969E-15,
0.996957691137886));
#43463=DIRECTION('center_axis',(4.88578148594761E-16,1.,1.17579033359749E-15));
#43464=DIRECTION('ref_axis',(0.0779446090567885,1.13413118345969E-15,-0.996957691137886));
#43465=DIRECTION('',(-4.88578148594761E-16,-1.,-1.17579033359749E-15));
#43466=DIRECTION('center_axis',(4.88578148594761E-16,1.,1.17579033359749E-15));
#43467=DIRECTION('ref_axis',(0.996957691137886,-5.78738260848462E-16,0.0779446090567885));
#43468=DIRECTION('',(-4.88578148594761E-16,-1.,-1.17579033359749E-15));
#43469=DIRECTION('',(4.88578148594761E-16,1.,1.17579033359749E-15));
#43470=DIRECTION('center_axis',(4.88578148594761E-16,1.,1.17579033359749E-15));
#43471=DIRECTION('ref_axis',(0.996957691137886,-5.78738260848462E-16,0.0779446090567885));
#43472=DIRECTION('center_axis',(-4.88578148594761E-16,-1.,-1.17579033359749E-15));
#43473=DIRECTION('ref_axis',(-0.0779446090567885,-1.13413118345969E-15,
0.996957691137886));
#43474=DIRECTION('center_axis',(4.88578148594761E-16,1.,1.17579033359749E-15));
#43475=DIRECTION('ref_axis',(-0.0779446090567885,-1.13413118345969E-15,
0.996957691137886));
#43476=DIRECTION('center_axis',(4.88578148594761E-16,1.,1.17579033359749E-15));
#43477=DIRECTION('ref_axis',(-0.0779446090567885,-1.13413118345969E-15,
0.996957691137886));
#43478=DIRECTION('',(-0.0551151616209889,0.707106781186552,0.704955543959679));
#43479=DIRECTION('center_axis',(-4.88578148594761E-16,-1.,-1.17579033359749E-15));
#43480=DIRECTION('ref_axis',(-0.0779446090567885,-1.13413118345969E-15,
0.996957691137886));
#43481=DIRECTION('center_axis',(4.88578148594761E-16,1.,1.17579033359749E-15));
#43482=DIRECTION('ref_axis',(0.0779446090567885,1.13413118345969E-15,-0.996957691137886));
#43483=DIRECTION('',(-4.88578148594761E-16,-1.,-1.17579033359749E-15));
#43484=DIRECTION('center_axis',(-4.88578148594761E-16,-1.,-1.17579033359749E-15));
#43485=DIRECTION('ref_axis',(-0.0779446090567887,-1.13413118345969E-15,
0.996957691137886));
#43486=DIRECTION('center_axis',(-4.88578148594761E-16,-1.,-1.17579033359749E-15));
#43487=DIRECTION('ref_axis',(-0.0779446090567887,-1.13413118345969E-15,
0.996957691137886));
#43488=DIRECTION('center_axis',(4.88578148594761E-16,1.,1.17579033359749E-15));
#43489=DIRECTION('ref_axis',(0.996957691137886,-5.78738260848462E-16,0.0779446090567885));
#43490=DIRECTION('center_axis',(0.996957691137886,-6.86676610464798E-16,
0.0779446090567885));
#43491=DIRECTION('ref_axis',(5.96188116413496E-16,1.,1.18420354606057E-15));
#43492=DIRECTION('',(-0.0779446090567885,-1.13413118345969E-15,0.996957691137886));
#43493=DIRECTION('',(5.96188116413496E-16,1.,1.18420354606057E-15));
#43494=DIRECTION('',(-0.0779446090567885,-1.13413118345969E-15,0.996957691137886));
#43495=DIRECTION('center_axis',(-0.0779446090567885,-1.13413118345969E-15,
0.996957691137886));
#43496=DIRECTION('ref_axis',(-5.18990262561707E-16,1.,1.09701615230207E-15));
#43497=DIRECTION('center_axis',(-0.0779446090567885,-1.13413118345969E-15,
0.996957691137886));
#43498=DIRECTION('ref_axis',(-4.8857814859476E-16,-1.,-1.17579033359749E-15));
#43499=DIRECTION('',(-0.0779446090567885,-1.13413118345969E-15,0.996957691137886));
#43500=DIRECTION('center_axis',(-0.996957691137886,8.41043700732428E-16,
-0.0779446090567885));
#43501=DIRECTION('ref_axis',(-7.50085574314386E-16,-1.,-1.19623562856271E-15));
#43502=DIRECTION('',(-6.19242119716166E-16,-1.,-1.18600596484984E-15));
#43503=DIRECTION('',(-0.0779446090567885,-1.13413118345969E-15,0.996957691137886));
#43504=DIRECTION('center_axis',(-0.0779446090567885,-1.13413118345969E-15,
0.996957691137886));
#43505=DIRECTION('ref_axis',(-4.88578148594761E-16,-1.,-1.17579033359749E-15));
#43506=DIRECTION('center_axis',(-0.0779446090567885,-1.13413118345969E-15,
0.996957691137886));
#43507=DIRECTION('ref_axis',(-4.88578148594761E-16,-1.,-1.17579033359749E-15));
#43508=DIRECTION('center_axis',(-0.0779446090567885,-1.13413118345969E-15,
0.996957691137886));
#43509=DIRECTION('ref_axis',(0.996957691137886,-5.78738260848462E-16,0.0779446090567885));
#43510=DIRECTION('center_axis',(4.88578148594761E-16,1.,1.17579033359749E-15));
#43511=DIRECTION('ref_axis',(-0.0779446090567885,-1.13413118345969E-15,
0.996957691137886));
#43512=DIRECTION('center_axis',(-4.88578148594761E-16,-1.,-1.17579033359749E-15));
#43513=DIRECTION('ref_axis',(-0.0779446090567885,-1.13413118345969E-15,
0.996957691137886));
#43514=DIRECTION('center_axis',(-4.88578148594761E-16,-1.,-1.17579033359749E-15));
#43515=DIRECTION('ref_axis',(-0.0779446090567885,-1.13413118345969E-15,
0.996957691137886));
#43516=DIRECTION('',(-0.0551151616209894,-0.707106781186553,0.704955543959677));
#43517=DIRECTION('center_axis',(4.88578148594761E-16,1.,1.17579033359749E-15));
#43518=DIRECTION('ref_axis',(-0.0779446090567885,-1.13413118345969E-15,
0.996957691137886));
#43519=DIRECTION('center_axis',(-4.88578148594761E-16,-1.,-1.17579033359749E-15));
#43520=DIRECTION('ref_axis',(-0.996957691137886,5.78738260848462E-16,-0.0779446090567885));
#43521=DIRECTION('center_axis',(-4.88578148594761E-16,-1.,-1.17579033359749E-15));
#43522=DIRECTION('ref_axis',(-0.0779446090567887,-1.13413118345969E-15,
0.996957691137886));
#43523=DIRECTION('center_axis',(4.88578148594761E-16,1.,1.17579033359749E-15));
#43524=DIRECTION('ref_axis',(0.0779446090567885,1.13413118345969E-15,-0.996957691137886));
#43525=DIRECTION('center_axis',(4.88578148594761E-16,1.,1.17579033359749E-15));
#43526=DIRECTION('ref_axis',(0.996957691137886,-5.78738260848463E-16,0.0779446090567885));
#43527=DIRECTION('',(-4.88578148594761E-16,-1.,-1.17579033359749E-15));
#43528=DIRECTION('center_axis',(4.88578148594761E-16,1.,1.17579033359749E-15));
#43529=DIRECTION('ref_axis',(0.996957691137886,-5.78738260848463E-16,0.0779446090567885));
#43530=DIRECTION('center_axis',(4.88578148594761E-16,1.,1.17579033359749E-15));
#43531=DIRECTION('ref_axis',(0.996957691137886,0.,0.0779446090567894));
#43532=DIRECTION('center_axis',(0.0779446090567902,1.13413118345969E-15,
-0.996957691137886));
#43533=DIRECTION('ref_axis',(-0.996957691137886,0.,-0.0779446090567902));
#43534=DIRECTION('center_axis',(4.88578148594761E-16,1.,1.17579033359749E-15));
#43535=DIRECTION('ref_axis',(-0.0779446090567887,-1.13413118345969E-15,
0.996957691137886));
#43536=DIRECTION('center_axis',(4.88578148594761E-16,1.,1.17579033359749E-15));
#43537=DIRECTION('ref_axis',(-0.0779446090567887,-1.13413118345969E-15,
0.996957691137886));
#43538=DIRECTION('center_axis',(4.88578148594761E-16,1.,1.17579033359749E-15));
#43539=DIRECTION('ref_axis',(0.0779446090567885,1.13413118345969E-15,-0.996957691137886));
#43540=DIRECTION('',(-4.88578148594761E-16,-1.,-1.17579033359749E-15));
#43541=DIRECTION('center_axis',(-4.88578148594761E-16,-1.,-1.17579033359749E-15));
#43542=DIRECTION('ref_axis',(-0.0779446090567885,-1.13413118345969E-15,
0.996957691137886));
#43543=DIRECTION('center_axis',(-4.88578148594761E-16,-1.,-1.17579033359749E-15));
#43544=DIRECTION('ref_axis',(-0.0779446090567885,-1.13413118345969E-15,
0.996957691137886));
#43545=DIRECTION('center_axis',(4.88578148594761E-16,1.,1.17579033359749E-15));
#43546=DIRECTION('ref_axis',(0.996957691137886,-8.88178419700125E-16,0.0779446090567894));
#43547=DIRECTION('center_axis',(0.0779446090567902,1.13413118345969E-15,
-0.996957691137886));
#43548=DIRECTION('ref_axis',(-0.996957691137886,1.11022302462515E-15,-0.0779446090567902));
#43549=DIRECTION('center_axis',(4.88578148594761E-16,1.,1.17579033359749E-15));
#43550=DIRECTION('ref_axis',(-0.0779446090567887,-1.13413118345969E-15,
0.996957691137886));
#43551=DIRECTION('center_axis',(4.88578148594761E-16,1.,1.17579033359749E-15));
#43552=DIRECTION('ref_axis',(0.996957691137886,-5.78738260848462E-16,0.0779446090567885));
#43553=DIRECTION('center_axis',(-4.88578148594761E-16,-1.,-1.17579033359749E-15));
#43554=DIRECTION('ref_axis',(-0.0779446090567885,-1.13413118345969E-15,
0.996957691137886));
#43555=DIRECTION('center_axis',(-4.88578148594761E-16,-1.,-1.17579033359749E-15));
#43556=DIRECTION('ref_axis',(-0.0779446090567885,-1.13413118345969E-15,
0.996957691137886));
#43557=DIRECTION('center_axis',(4.88578148594761E-16,1.,1.17579033359749E-15));
#43558=DIRECTION('ref_axis',(-0.0779446090567885,-1.13413118345969E-15,
0.996957691137886));
#43559=DIRECTION('center_axis',(4.88578148594761E-16,1.,1.17579033359749E-15));
#43560=DIRECTION('ref_axis',(-0.0779446090567885,-1.13413118345969E-15,
0.996957691137886));
#43561=DIRECTION('',(-0.0551151616209894,0.707106781186545,0.704955543959685));
#43562=DIRECTION('center_axis',(4.88578148594761E-16,1.,1.17579033359749E-15));
#43563=DIRECTION('ref_axis',(0.0779446090567885,1.13413118345969E-15,-0.996957691137886));
#43564=DIRECTION('',(-4.88578148594761E-16,-1.,-1.17579033359749E-15));
#43565=DIRECTION('center_axis',(4.88578148594761E-16,1.,1.17579033359749E-15));
#43566=DIRECTION('ref_axis',(0.996957691137886,-5.78738260848463E-16,0.0779446090567885));
#43567=DIRECTION('center_axis',(4.88578148594761E-16,1.,1.17579033359749E-15));
#43568=DIRECTION('ref_axis',(0.996957691137886,-5.78738260848463E-16,0.0779446090567885));
#43569=DIRECTION('center_axis',(4.88578148594761E-16,1.,1.17579033359749E-15));
#43570=DIRECTION('ref_axis',(-0.0779446090567885,-1.13413118345969E-15,
0.996957691137886));
#43571=DIRECTION('',(-0.0551151616209896,-0.707106781186551,0.70495554395968));
#43572=DIRECTION('center_axis',(4.88578148594761E-16,1.,1.17579033359749E-15));
#43573=DIRECTION('ref_axis',(-0.0779446090567885,-1.13413118345969E-15,
0.996957691137886));
#43574=DIRECTION('center_axis',(-4.88578148594761E-16,-1.,-1.17579033359749E-15));
#43575=DIRECTION('ref_axis',(-0.996957691137886,5.78738260848462E-16,-0.0779446090567885));
#43576=DIRECTION('center_axis',(-0.0779446090567885,-1.13413118345969E-15,
0.996957691137886));
#43577=DIRECTION('ref_axis',(0.996957691137886,-5.78738260848462E-16,0.0779446090567885));
#43578=DIRECTION('',(-0.0779446090567885,-1.13413118345969E-15,0.996957691137886));
#43579=DIRECTION('center_axis',(-0.0779446090567885,-1.13413118345969E-15,
0.996957691137886));
#43580=DIRECTION('ref_axis',(0.996957691137886,-5.78738260848462E-16,0.0779446090567885));
#43581=DIRECTION('',(-0.0779446090567885,-1.13413118345969E-15,0.996957691137886));
#43582=DIRECTION('center_axis',(0.996957691137886,-5.78738260848463E-16,
0.0779446090567885));
#43583=DIRECTION('ref_axis',(4.88578148594761E-16,1.,1.17579033359749E-15));
#43584=DIRECTION('',(4.88578148594761E-16,1.,1.17579033359749E-15));
#43585=DIRECTION('',(4.88578148594761E-16,1.,1.17579033359749E-15));
#43586=DIRECTION('',(-0.0779446090567885,-1.13413118345969E-15,0.996957691137886));
#43587=DIRECTION('center_axis',(-0.996957691137886,5.78738260848463E-16,
-0.0779446090567885));
#43588=DIRECTION('ref_axis',(-4.88578148594761E-16,-1.,-1.17579033359749E-15));
#43589=DIRECTION('',(-0.0779446090567885,-1.13413118345969E-15,0.996957691137886));
#43590=DIRECTION('',(-4.88578148594761E-16,-1.,-1.17579033359749E-15));
#43591=DIRECTION('center_axis',(-0.0779446090567885,-1.13413118345969E-15,
0.996957691137886));
#43592=DIRECTION('ref_axis',(-0.996957691137886,5.78738260848462E-16,-0.0779446090567885));
#43593=DIRECTION('center_axis',(-0.0779446090567885,-1.13413118345969E-15,
0.996957691137886));
#43594=DIRECTION('ref_axis',(-0.996957691137886,5.78738260848462E-16,-0.0779446090567885));
#43595=DIRECTION('center_axis',(0.0779446090567885,1.13413118345969E-15,
-0.996957691137886));
#43596=DIRECTION('ref_axis',(-0.996957691137886,5.78738260848462E-16,-0.0779446090567885));
#43597=DIRECTION('center_axis',(4.88578148594761E-16,1.,1.17579033359749E-15));
#43598=DIRECTION('ref_axis',(0.0779446090567885,1.13413118345969E-15,-0.996957691137886));
#43599=DIRECTION('center_axis',(4.88578148594761E-16,1.,1.17579033359749E-15));
#43600=DIRECTION('ref_axis',(0.996957691137886,-5.78738260848463E-16,0.0779446090567885));
#43601=DIRECTION('center_axis',(4.88578148594761E-16,1.,1.17579033359749E-15));
#43602=DIRECTION('ref_axis',(0.996957691137886,-5.78738260848463E-16,0.0779446090567885));
#43603=DIRECTION('center_axis',(4.88578148594761E-16,1.,1.17579033359749E-15));
#43604=DIRECTION('ref_axis',(0.996957691137886,0.,0.0779446090567891));
#43605=DIRECTION('center_axis',(4.88578148594761E-16,1.,1.17579033359749E-15));
#43606=DIRECTION('ref_axis',(0.996957691137886,-5.78738260848463E-16,0.0779446090567885));
#43607=DIRECTION('center_axis',(0.0779446090567875,1.13413118345969E-15,
-0.996957691137886));
#43608=DIRECTION('ref_axis',(-0.996957691137886,0.,-0.0779446090567875));
#43609=DIRECTION('center_axis',(-4.88578148594761E-16,-1.,-1.17579033359749E-15));
#43610=DIRECTION('ref_axis',(-0.996957691137886,5.78738260848462E-16,-0.0779446090567885));
#43611=DIRECTION('center_axis',(4.88578148594761E-16,1.,1.17579033359749E-15));
#43612=DIRECTION('ref_axis',(0.996957691137886,-5.78738260848463E-16,0.0779446090567885));
#43613=DIRECTION('center_axis',(4.88578148594761E-16,1.,1.17579033359749E-15));
#43614=DIRECTION('ref_axis',(0.0779446090567885,1.13413118345969E-15,-0.996957691137886));
#43615=DIRECTION('',(0.0551151616209892,-0.707106781186546,-0.704955543959685));
#43616=DIRECTION('center_axis',(-4.88578148594761E-16,-1.,-1.17579033359749E-15));
#43617=DIRECTION('ref_axis',(0.0779446090567885,1.13413118345969E-15,-0.996957691137886));
#43618=DIRECTION('',(0.0551151616209901,0.707106781186547,-0.704955543959683));
#43619=DIRECTION('center_axis',(4.88578148594761E-16,1.,1.17579033359749E-15));
#43620=DIRECTION('ref_axis',(0.996957691137886,-5.78738260848463E-16,0.0779446090567885));
#43621=DIRECTION('center_axis',(4.88578148594761E-16,1.,1.17579033359749E-15));
#43622=DIRECTION('ref_axis',(0.996957691137886,-5.78738260848462E-16,0.0779446090567885));
#43623=DIRECTION('center_axis',(4.88578148594761E-16,1.,1.17579033359749E-15));
#43624=DIRECTION('ref_axis',(0.996957691137886,-5.78738260848463E-16,0.0779446090567885));
#43625=DIRECTION('center_axis',(4.88578148594761E-16,1.,1.17579033359749E-15));
#43626=DIRECTION('ref_axis',(0.996957691137886,-7.28761780266769E-16,0.0779446090567891));
#43627=DIRECTION('center_axis',(0.0779446090567878,1.13413118345969E-15,
-0.996957691137886));
#43628=DIRECTION('ref_axis',(-0.996957691137886,9.10952225333462E-16,-0.0779446090567878));
#56106=CARTESIAN_POINT('',(0.,0.,0.));
#56107=CARTESIAN_POINT('Origin',(375.115917770968,-180.47200726879,445.000000551892));
#56108=CARTESIAN_POINT('',(373.557025589832,-105.97200726879,464.93915437465));
#56109=CARTESIAN_POINT('',(373.557025589832,-254.972007268791,464.93915437465));
#56110=CARTESIAN_POINT('',(373.557025589832,-180.47200726879,464.93915437465));
#56111=CARTESIAN_POINT('',(376.674809952104,-105.97200726879,425.060846729135));
#56112=CARTESIAN_POINT('Origin',(375.115917770968,-105.97200726879,445.000000551892));
#56113=CARTESIAN_POINT('',(370.621259986509,-111.97200726879,425.511592422941));
#56114=CARTESIAN_POINT('Ctrl Pts',(376.674809952104,-105.97200726879,425.060846729135));
#56115=CARTESIAN_POINT('Ctrl Pts',(375.918788491129,-105.97200726879,425.001739108282));
#56116=CARTESIAN_POINT('Ctrl Pts',(375.111798551165,-106.124510775769,424.986188615741));
#56117=CARTESIAN_POINT('Ctrl Pts',(373.625980083073,-106.738309454724,425.041724802303));
#56118=CARTESIAN_POINT('Ctrl Pts',(372.946965023565,-107.199354583986,425.110561308361));
#56119=CARTESIAN_POINT('Ctrl Pts',(371.872070611148,-108.259536519781,425.257361914111));
#56120=CARTESIAN_POINT('Ctrl Pts',(371.402882122954,-108.931056193358,425.345094021509));
#56121=CARTESIAN_POINT('Ctrl Pts',(370.777249287815,-110.407792297934,425.473660795511));
#56122=CARTESIAN_POINT('Ctrl Pts',(370.621259986509,-111.213452760812,425.511592422941));
#56123=CARTESIAN_POINT('Ctrl Pts',(370.621259986509,-111.97200726879,425.511592422941));
#56124=CARTESIAN_POINT('',(370.621259986508,-248.97200726879,425.51159242294));
#56125=CARTESIAN_POINT('',(370.621259986508,-180.47200726879,425.511592422941));
#56126=CARTESIAN_POINT('',(376.674809952104,-254.97200726879,425.060846729135));
#56127=CARTESIAN_POINT('Ctrl Pts',(370.621259986508,-248.97200726879,425.51159242294));
#56128=CARTESIAN_POINT('Ctrl Pts',(370.621259986508,-249.730561776769,425.51159242294));
#56129=CARTESIAN_POINT('Ctrl Pts',(370.777249287815,-250.536222239647,425.473660795511));
#56130=CARTESIAN_POINT('Ctrl Pts',(371.402882122954,-252.012958344223,425.345094021508));
#56131=CARTESIAN_POINT('Ctrl Pts',(371.872070611148,-252.6844780178,425.257361914111));
#56132=CARTESIAN_POINT('Ctrl Pts',(372.946965023565,-253.744659953595,425.110561308361));
#56133=CARTESIAN_POINT('Ctrl Pts',(373.625980083073,-254.205705082856,425.041724802303));
#56134=CARTESIAN_POINT('Ctrl Pts',(375.111798551165,-254.819503761812,424.98618861574));
#56135=CARTESIAN_POINT('Ctrl Pts',(375.918788491129,-254.97200726879,425.001739108282));
#56136=CARTESIAN_POINT('Ctrl Pts',(376.674809952104,-254.97200726879,425.060846729135));
#56137=CARTESIAN_POINT('Origin',(375.115917770968,-254.97200726879,445.000000551892));
#56138=CARTESIAN_POINT('Origin',(375.115917770968,70.2779927312095,445.000000551893));
#56139=CARTESIAN_POINT('',(376.090225384178,70.0279927312094,432.538029412669));
#56140=CARTESIAN_POINT('',(374.141610157758,70.0279927312094,457.461971691116));
#56141=CARTESIAN_POINT('Origin',(375.115917770968,70.0279927312094,445.000000551893));
#56142=CARTESIAN_POINT('Origin',(375.115917770968,70.0279927312094,445.000000551893));
#56143=CARTESIAN_POINT('',(376.05125307965,70.5279927312094,433.036508258238));
#56144=CARTESIAN_POINT('',(376.070739231914,70.2779927312095,432.787268835454));
#56145=CARTESIAN_POINT('Origin',(375.115917770968,70.5279927312094,445.000000551893));
#56146=CARTESIAN_POINT('Origin',(375.115917770968,20.5279927312094,445.000000551893));
#56147=CARTESIAN_POINT('',(374.141610157758,-29.4720072687906,457.461971691116));
#56148=CARTESIAN_POINT('',(374.141610157758,20.5279927312094,457.461971691116));
#56149=CARTESIAN_POINT('Origin',(375.115917770968,-29.4720072687906,445.000000551893));
#56150=CARTESIAN_POINT('',(369.988900990807,56.9410394849244,433.599838319014));
#56151=CARTESIAN_POINT('',(369.988900990807,-15.0589605150756,433.599838319014));
#56152=CARTESIAN_POINT('',(369.988900990807,20.5279927312094,433.599838319014));
#56153=CARTESIAN_POINT('',(381.952393284462,-15.0589605150756,434.535173627696));
#56154=CARTESIAN_POINT('Ctrl Pts',(369.988900990807,-15.0589605150755,433.599838319014));
#56155=CARTESIAN_POINT('Ctrl Pts',(369.988900990807,-15.8272357942547,433.599838319014));
#56156=CARTESIAN_POINT('Ctrl Pts',(370.151524843035,-16.635872857665,433.522949429245));
#56157=CARTESIAN_POINT('Ctrl Pts',(370.78905122987,-18.1091493532521,433.267732479884));
#56158=CARTESIAN_POINT('Ctrl Pts',(371.263063224569,-18.7752122333175,433.095435318238));
#56159=CARTESIAN_POINT('Ctrl Pts',(372.341025514289,-19.8267981076742,432.799110512512));
#56160=CARTESIAN_POINT('Ctrl Pts',(373.020881601515,-20.2868198879197,432.653987167789));
#56161=CARTESIAN_POINT('Ctrl Pts',(374.513080057484,-20.9032184113205,432.492010706903));
#56162=CARTESIAN_POINT('Ctrl Pts',(375.326021983044,-21.0589605150756,432.478282107572));
#56163=CARTESIAN_POINT('Ctrl Pts',(376.854428785312,-21.0589605150756,432.597776717766));
#56164=CARTESIAN_POINT('Ctrl Pts',(377.655359248128,-20.9032184113205,432.737681837422));
#56165=CARTESIAN_POINT('Ctrl Pts',(379.104252847889,-20.2868198879197,433.129600122843));
#56166=CARTESIAN_POINT('Ctrl Pts',(379.753293853246,-19.8267981076742,433.378619917013));
#56167=CARTESIAN_POINT('Ctrl Pts',(380.77210481419,-18.7752122333175,433.838875622472));
#56168=CARTESIAN_POINT('Ctrl Pts',(381.213579664274,-18.1091493532521,434.082747801641));
#56169=CARTESIAN_POINT('Ctrl Pts',(381.803695113145,-16.635872857665,434.433944814947));
#56170=CARTESIAN_POINT('Ctrl Pts',(381.952393284462,-15.8272357942547,434.535173627696));
#56171=CARTESIAN_POINT('Ctrl Pts',(381.952393284462,-15.0589605150756,434.535173627696));
#56172=CARTESIAN_POINT('',(381.952393284462,56.9410394849244,434.535173627696));
#56173=CARTESIAN_POINT('',(381.952393284462,20.5279927312094,434.535173627696));
#56174=CARTESIAN_POINT('Ctrl Pts',(381.952393284462,56.9410394849244,434.535173627696));
#56175=CARTESIAN_POINT('Ctrl Pts',(381.952393284462,57.7093147641036,434.535173627696));
#56176=CARTESIAN_POINT('Ctrl Pts',(381.803695113145,58.5179518275139,434.433944814947));
#56177=CARTESIAN_POINT('Ctrl Pts',(381.213579664274,59.991228323101,434.082747801641));
#56178=CARTESIAN_POINT('Ctrl Pts',(380.77210481419,60.6572912031664,433.838875622472));
#56179=CARTESIAN_POINT('Ctrl Pts',(379.753293853246,61.7088770775231,433.378619917013));
#56180=CARTESIAN_POINT('Ctrl Pts',(379.104252847889,62.1688988577686,433.129600122844));
#56181=CARTESIAN_POINT('Ctrl Pts',(377.655359248128,62.7852973811694,432.737681837422));
#56182=CARTESIAN_POINT('Ctrl Pts',(376.854428785312,62.9410394849244,432.597776717766));
#56183=CARTESIAN_POINT('Ctrl Pts',(375.326021983044,62.9410394849244,432.478282107572));
#56184=CARTESIAN_POINT('Ctrl Pts',(374.513080057484,62.7852973811694,432.492010706903));
#56185=CARTESIAN_POINT('Ctrl Pts',(373.020881601515,62.1688988577686,432.65398716779));
#56186=CARTESIAN_POINT('Ctrl Pts',(372.341025514289,61.7088770775231,432.799110512512));
#56187=CARTESIAN_POINT('Ctrl Pts',(371.263063224569,60.6572912031664,433.095435318238));
#56188=CARTESIAN_POINT('Ctrl Pts',(370.78905122987,59.991228323101,433.267732479884));
#56189=CARTESIAN_POINT('Ctrl Pts',(370.151524843035,58.5179518275139,433.522949429245));
#56190=CARTESIAN_POINT('Ctrl Pts',(369.988900990807,57.7093147641036,433.599838319014));
#56191=CARTESIAN_POINT('Ctrl Pts',(369.988900990807,56.9410394849244,433.599838319014));
#56192=CARTESIAN_POINT('Origin',(375.115917770968,70.5279927312094,445.000000551893));
#56193=CARTESIAN_POINT('Origin',(375.115917770968,-29.7220072687906,445.000000551893));
#56194=CARTESIAN_POINT('',(376.28508690682,-29.9720072687906,430.045635184824));
#56195=CARTESIAN_POINT('',(373.946748635116,-29.9720072687906,459.954365918961));
#56196=CARTESIAN_POINT('Origin',(375.115917770968,-29.9720072687906,445.000000551893));
#56197=CARTESIAN_POINT('Origin',(375.115917770968,-29.9720072687906,445.000000551893));
#56198=CARTESIAN_POINT('',(376.246114602291,-29.4720072687906,430.544114030393));
#56199=CARTESIAN_POINT('',(376.265600754556,-29.7220072687906,430.294874607609));
#56200=CARTESIAN_POINT('Origin',(375.115917770968,-29.4720072687906,445.000000551893));
#56201=CARTESIAN_POINT('Origin',(375.115917770968,-62.3557281990226,445.000000551893));
#56202=CARTESIAN_POINT('',(373.946748635116,-98.9720072687905,459.954365918961));
#56203=CARTESIAN_POINT('',(373.946748635116,-62.3557281990226,459.954365918961));
#56204=CARTESIAN_POINT('',(360.1615524039,-98.9720072687905,443.830831416041));
#56205=CARTESIAN_POINT('Origin',(375.115917770968,-98.9720072687905,445.000000551892));
#56206=CARTESIAN_POINT('Origin',(375.115917770968,-98.9720072687905,445.000000551892));
#56207=CARTESIAN_POINT('Origin',(376.090225384178,-29.4720072687906,432.538029412669));
#56208=CARTESIAN_POINT('Origin',(382.266833053647,-15.0589605150756,430.513302839165));
#56209=CARTESIAN_POINT('',(381.643276181193,-15.0589605150756,438.488964368268));
#56210=CARTESIAN_POINT('',(382.266833053647,-15.0589605150756,430.513302839165));
#56211=CARTESIAN_POINT('',(381.643276181193,56.9410394849244,438.488964368268));
#56212=CARTESIAN_POINT('',(381.643276181193,56.9410394849244,438.488964368268));
#56213=CARTESIAN_POINT('',(382.266833053647,56.9410394849244,430.513302839165));
#56214=CARTESIAN_POINT('Origin',(376.28508690682,56.9410394849244,430.045635184824));
#56215=CARTESIAN_POINT('',(369.679783887538,56.9410394849244,437.553629059587));
#56216=CARTESIAN_POINT('Origin',(375.661530034366,56.9410394849244,438.021296713927));
#56217=CARTESIAN_POINT('',(370.303340759993,56.9410394849244,429.577967530484));
#56218=CARTESIAN_POINT('Origin',(370.303340759993,-10.8264023755406,429.577967530484));
#56219=CARTESIAN_POINT('',(369.679783887538,-15.0589605150756,437.553629059587));
#56220=CARTESIAN_POINT('',(369.679783887538,-10.8264023755406,437.553629059587));
#56221=CARTESIAN_POINT('',(370.303340759993,-15.0589605150756,429.577967530484));
#56222=CARTESIAN_POINT('Origin',(376.28508690682,-15.0589605150756,430.045635184824));
#56223=CARTESIAN_POINT('Origin',(375.661530034366,-15.0589605150756,438.021296713927));
#56224=CARTESIAN_POINT('Origin',(375.661530034366,-15.0589605150756,438.021296713927));
#56225=CARTESIAN_POINT('Origin',(375.115917770968,-260.72200726879,445.000000551892));
#56226=CARTESIAN_POINT('',(376.557893038519,-260.47200726879,426.556283265841));
#56227=CARTESIAN_POINT('',(373.673942503417,-260.47200726879,463.443717837943));
#56228=CARTESIAN_POINT('Origin',(375.115917770968,-260.47200726879,445.000000551892));
#56229=CARTESIAN_POINT('Origin',(375.115917770968,-260.47200726879,445.000000551892));
#56230=CARTESIAN_POINT('',(376.51892073399,-260.97200726879,427.05476211141));
#56231=CARTESIAN_POINT('',(376.538406886254,-260.72200726879,426.805522688626));
#56232=CARTESIAN_POINT('Origin',(375.115917770968,-260.97200726879,445.000000551892));
#56233=CARTESIAN_POINT('Origin',(376.557893038519,-260.97200726879,426.556283265841));
#56234=CARTESIAN_POINT('',(359.663073558331,-260.97200726879,443.791859111512));
#56235=CARTESIAN_POINT('Origin',(375.115917770968,-260.97200726879,445.000000551892));
#56236=CARTESIAN_POINT('Origin',(375.115917770968,-258.47200726879,445.000000551892));
#56237=CARTESIAN_POINT('',(373.673942503417,-255.972007268791,463.443717837943));
#56238=CARTESIAN_POINT('',(356.672200484917,-255.97200726879,443.558025284342));
#56239=CARTESIAN_POINT('Origin',(375.115917770968,-255.97200726879,445.000000551892));
#56240=CARTESIAN_POINT('',(373.673942503417,-258.472007268791,463.443717837943));
#56241=CARTESIAN_POINT('Origin',(375.115917770968,-255.97200726879,445.000000551892));
#56242=CARTESIAN_POINT('Origin',(375.115917770968,-261.47200726879,445.000000551892));
#56243=CARTESIAN_POINT('',(360.1615524039,-261.47200726879,443.83083141604));
#56244=CARTESIAN_POINT('Origin',(359.663073558331,-261.47200726879,443.791859111512));
#56245=CARTESIAN_POINT('',(373.946748635116,-261.47200726879,459.954365918961));
#56246=CARTESIAN_POINT('Origin',(375.115917770968,-261.47200726879,445.000000551892));
#56247=CARTESIAN_POINT('Origin',(375.115917770968,-261.47200726879,445.000000551892));
#56248=CARTESIAN_POINT('Origin',(375.115917770968,-295.972007268791,445.000000551892));
#56249=CARTESIAN_POINT('',(373.946748635116,-329.972007268791,459.95436591896));
#56250=CARTESIAN_POINT('',(373.946748635116,-295.972007268791,459.954365918961));
#56251=CARTESIAN_POINT('',(376.28508690682,-329.972007268791,430.045635184824));
#56252=CARTESIAN_POINT('Origin',(375.115917770968,-329.972007268791,445.000000551892));
#56253=CARTESIAN_POINT('Origin',(375.115917770968,-329.972007268791,445.000000551892));
#56254=CARTESIAN_POINT('Origin',(375.115917770968,-98.9720072687905,445.000000551892));
#56255=CARTESIAN_POINT('',(359.663073558331,-99.4720072687904,443.791859111512));
#56256=CARTESIAN_POINT('Origin',(359.663073558331,-98.9720072687905,443.791859111512));
#56257=CARTESIAN_POINT('Origin',(375.115917770968,-99.4720072687905,445.000000551892));
#56258=CARTESIAN_POINT('Origin',(376.28508690682,-99.4720072687905,430.045635184824));
#56259=CARTESIAN_POINT('',(376.51892073399,-99.4720072687905,427.054762111411));
#56260=CARTESIAN_POINT('Origin',(375.115917770968,-99.4720072687905,445.000000551892));
#56261=CARTESIAN_POINT('Origin',(375.115917770968,-99.7220072687905,445.000000551892));
#56262=CARTESIAN_POINT('',(376.557893038519,-99.9720072687904,426.556283265842));
#56263=CARTESIAN_POINT('',(373.673942503417,-99.9720072687905,463.443717837943));
#56264=CARTESIAN_POINT('Origin',(375.115917770968,-99.9720072687905,445.000000551892));
#56265=CARTESIAN_POINT('Origin',(375.115917770968,-99.9720072687905,445.000000551892));
#56266=CARTESIAN_POINT('',(376.538406886254,-99.7220072687905,426.805522688626));
#56267=CARTESIAN_POINT('Origin',(375.115917770968,-102.22200726879,445.000000551892));
#56268=CARTESIAN_POINT('',(373.673942503417,-104.97200726879,463.443717837943));
#56269=CARTESIAN_POINT('',(373.673942503417,-102.222007268791,463.443717837943));
#56270=CARTESIAN_POINT('',(356.672200484917,-104.97200726879,443.558025284342));
#56271=CARTESIAN_POINT('Origin',(375.115917770968,-104.97200726879,445.000000551892));
#56272=CARTESIAN_POINT('Origin',(375.115917770968,-104.97200726879,445.000000551892));
#56273=CARTESIAN_POINT('Origin',(375.115917770968,-330.472007268791,445.000000551892));
#56274=CARTESIAN_POINT('',(376.207142297763,-330.972007268791,431.042592875962));
#56275=CARTESIAN_POINT('',(376.246114602291,-330.472007268791,430.544114030393));
#56276=CARTESIAN_POINT('Origin',(375.115917770968,-330.972007268791,445.000000551892));
#56277=CARTESIAN_POINT('Origin',(376.28508690682,-330.972007268791,430.045635184824));
#56278=CARTESIAN_POINT('Origin',(376.674809952104,-248.97200726879,425.060846729135));
#56279=CARTESIAN_POINT('',(370.069506932822,-248.97200726879,432.568840603897));
#56280=CARTESIAN_POINT('',(370.693063805276,-248.97200726879,424.593179074794));
#56281=CARTESIAN_POINT('',(382.032999226477,-248.97200726879,433.504175912578));
#56282=CARTESIAN_POINT('Origin',(376.051253079649,-248.97200726879,433.036508258238));
#56283=CARTESIAN_POINT('',(382.584752280163,-248.97200726879,426.446927731622));
#56284=CARTESIAN_POINT('',(382.656556098931,-248.97200726879,425.528514383475));
#56285=CARTESIAN_POINT('Ctrl Pts',(376.674809952104,-254.97200726879,425.060846729135));
#56286=CARTESIAN_POINT('Ctrl Pts',(377.430831413079,-254.97200726879,425.119954349988));
#56287=CARTESIAN_POINT('Ctrl Pts',(378.230432619979,-254.819503761812,425.230011112368));
#56288=CARTESIAN_POINT('Ctrl Pts',(379.689566163776,-254.205705082856,425.515790904349));
#56289=CARTESIAN_POINT('Ctrl Pts',(380.349632476106,-253.744659953595,425.689320091902));
#56290=CARTESIAN_POINT('Ctrl Pts',(381.388651133482,-252.6844780178,426.001391630682));
#56291=CARTESIAN_POINT('Ctrl Pts',(381.838503760257,-252.012958344223,426.160976637205));
#56292=CARTESIAN_POINT('Ctrl Pts',(382.436553503998,-250.536222239647,426.385213930697));
#56293=CARTESIAN_POINT('Ctrl Pts',(382.584752280163,-249.730561776769,426.446927731622));
#56294=CARTESIAN_POINT('Ctrl Pts',(382.584752280163,-248.97200726879,426.446927731622));
#56295=CARTESIAN_POINT('Origin',(382.656556098931,-248.97200726879,425.528514383475));
#56296=CARTESIAN_POINT('',(382.584752280163,-111.97200726879,426.446927731622));
#56297=CARTESIAN_POINT('',(382.584752280163,-180.47200726879,426.446927731622));
#56298=CARTESIAN_POINT('',(382.032999226477,-111.97200726879,433.504175912579));
#56299=CARTESIAN_POINT('',(382.032999226477,-111.97200726879,433.504175912579));
#56300=CARTESIAN_POINT('',(382.656556098931,-111.97200726879,425.528514383475));
#56301=CARTESIAN_POINT('Origin',(370.693063805276,-111.97200726879,424.593179074794));
#56302=CARTESIAN_POINT('',(370.069506932822,-111.97200726879,432.568840603897));
#56303=CARTESIAN_POINT('',(370.693063805276,-111.97200726879,424.593179074794));
#56304=CARTESIAN_POINT('',(370.069506932822,-248.97200726879,432.568840603897));
#56305=CARTESIAN_POINT('Origin',(376.674809952104,-111.97200726879,425.060846729135));
#56306=CARTESIAN_POINT('Ctrl Pts',(382.584752280163,-111.97200726879,426.446927731622));
#56307=CARTESIAN_POINT('Ctrl Pts',(382.584752280163,-111.213452760812,426.446927731622));
#56308=CARTESIAN_POINT('Ctrl Pts',(382.436553503998,-110.407792297934,426.385213930697));
#56309=CARTESIAN_POINT('Ctrl Pts',(381.838503760257,-108.931056193358,426.160976637205));
#56310=CARTESIAN_POINT('Ctrl Pts',(381.388651133482,-108.259536519781,426.001391630682));
#56311=CARTESIAN_POINT('Ctrl Pts',(380.349632476106,-107.199354583986,425.689320091903));
#56312=CARTESIAN_POINT('Ctrl Pts',(379.689566163776,-106.738309454725,425.51579090435));
#56313=CARTESIAN_POINT('Ctrl Pts',(378.230432619979,-106.124510775769,425.230011112368));
#56314=CARTESIAN_POINT('Ctrl Pts',(377.430831413079,-105.97200726879,425.119954349988));
#56315=CARTESIAN_POINT('Ctrl Pts',(376.674809952104,-105.97200726879,425.060846729135));
#56316=CARTESIAN_POINT('Origin',(376.051253079649,-111.97200726879,433.036508258238));
#56317=CARTESIAN_POINT('Origin',(376.051253079649,-180.47200726879,433.036508258238));
#56318=CARTESIAN_POINT('Origin',(375.115917770968,-180.47200726879,445.000000551892));
#56319=CARTESIAN_POINT('Origin',(375.115917770968,-254.97200726879,445.000000551892));
#56320=CARTESIAN_POINT('Origin',(375.115917770968,-105.97200726879,445.000000551892));
#56321=CARTESIAN_POINT('Origin',(375.115917770968,-255.97200726879,445.000000551892));
#56322=CARTESIAN_POINT('',(356.173721639348,-255.47200726879,443.519052979813));
#56323=CARTESIAN_POINT('Origin',(375.115917770968,-255.47200726879,445.000000551892));
#56324=CARTESIAN_POINT('Origin',(356.173721639348,-255.97200726879,443.519052979813));
#56325=CARTESIAN_POINT('Origin',(376.635837647575,-255.47200726879,425.559325574704));
#56326=CARTESIAN_POINT('',(373.595997894361,-255.472007268791,464.440675529081));
#56327=CARTESIAN_POINT('Origin',(375.115917770968,-255.47200726879,445.000000551892));
#56328=CARTESIAN_POINT('Origin',(375.115917770968,-255.22200726879,445.000000551892));
#56329=CARTESIAN_POINT('',(373.576511742096,-255.222007268791,464.689914951866));
#56330=CARTESIAN_POINT('Origin',(375.115917770968,-105.72200726879,445.000000551892));
#56331=CARTESIAN_POINT('',(373.595997894361,-105.47200726879,464.440675529081));
#56332=CARTESIAN_POINT('',(373.576511742096,-105.72200726879,464.689914951866));
#56333=CARTESIAN_POINT('Origin',(375.115917770968,-105.47200726879,445.000000551892));
#56334=CARTESIAN_POINT('Origin',(376.596865343047,-105.47200726879,426.057804420273));
#56335=CARTESIAN_POINT('',(356.173721639348,-105.47200726879,443.519052979813));
#56336=CARTESIAN_POINT('Origin',(375.115917770968,-105.47200726879,445.000000551892));
#56337=CARTESIAN_POINT('Origin',(375.115917770968,-104.97200726879,445.000000551892));
#56338=CARTESIAN_POINT('Origin',(356.173721639348,-104.97200726879,443.519052979813));
#61771=UNCERTAINTY_MEASURE_WITH_UNIT(LENGTH_MEASURE(0.01),#61812,
'DISTANCE_ACCURACY_VALUE',
'Maximum model space distance between geometric entities at asserted c
onnectivities');
#61780=UNCERTAINTY_MEASURE_WITH_UNIT(LENGTH_MEASURE(0.01),#61812,
'DISTANCE_ACCURACY_VALUE',
'Maximum model space distance between geometric entities at asserted c
onnectivities');
#61802=(
GEOMETRIC_REPRESENTATION_CONTEXT(3)
GLOBAL_UNCERTAINTY_ASSIGNED_CONTEXT((#61771))
GLOBAL_UNIT_ASSIGNED_CONTEXT((#61812,#61814,#61815))
REPRESENTATION_CONTEXT('','3D')
);
#61811=(
GEOMETRIC_REPRESENTATION_CONTEXT(3)
GLOBAL_UNCERTAINTY_ASSIGNED_CONTEXT((#61780))
GLOBAL_UNIT_ASSIGNED_CONTEXT((#61812,#61814,#61815))
REPRESENTATION_CONTEXT('','3D')
);
#61812=(
LENGTH_UNIT()
NAMED_UNIT(*)
SI_UNIT(.MILLI.,.METRE.)
);
#61814=(
NAMED_UNIT(*)
PLANE_ANGLE_UNIT()
SI_UNIT($,.RADIAN.)
);
#61815=(
NAMED_UNIT(*)
SI_UNIT($,.STERADIAN.)
SOLID_ANGLE_UNIT()
);
#61837=SHAPE_DEFINITION_REPRESENTATION(#61883,#61989);
#61883=PRODUCT_DEFINITION_SHAPE('',$,#62020);
#61989=SHAPE_REPRESENTATION('',(#36032),#61802);
#61998=PRODUCT_DEFINITION_CONTEXT('part definition',#62090,'design');
#62020=PRODUCT_DEFINITION('Cutter Shaft B','Cutter Shaft B',#62050,#61998);
#62050=PRODUCT_DEFINITION_FORMATION('',$,#62113);
#62090=APPLICATION_CONTEXT('Managed model based 3d engineering');
#62091=PRODUCT_CONTEXT('part definition',#62090,'mechanical');
#62113=PRODUCT('Cutter Shaft B','Cutter Shaft B',$,(#62091));
#62150=COLOUR_RGB('Grey',0.48,0.52,0.57);
#62151=FILL_AREA_STYLE_COLOUR('',#62150);
#62152=FILL_AREA_STYLE('',(#62151));
#62153=SURFACE_STYLE_FILL_AREA(#62152);
#62154=SURFACE_SIDE_STYLE('',(#62153));
#62155=SURFACE_STYLE_USAGE(.BOTH.,#62154);
#62156=PRESENTATION_STYLE_ASSIGNMENT((#62155));
ENDSEC;
END-ISO-10303-21;
